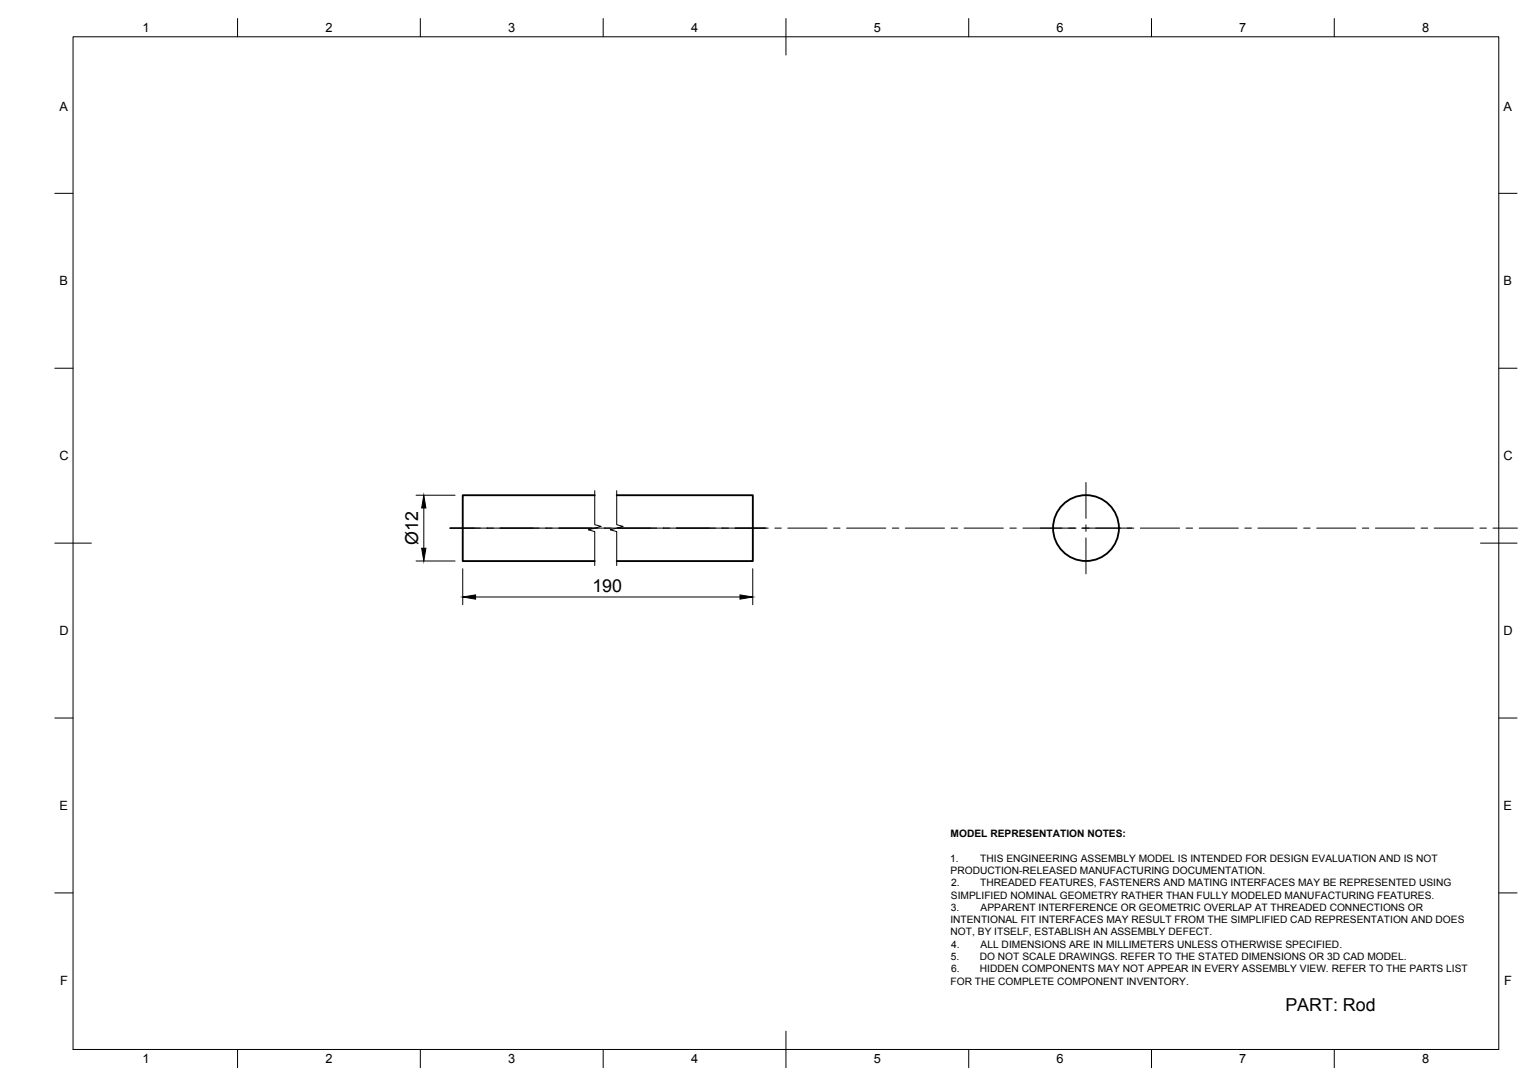
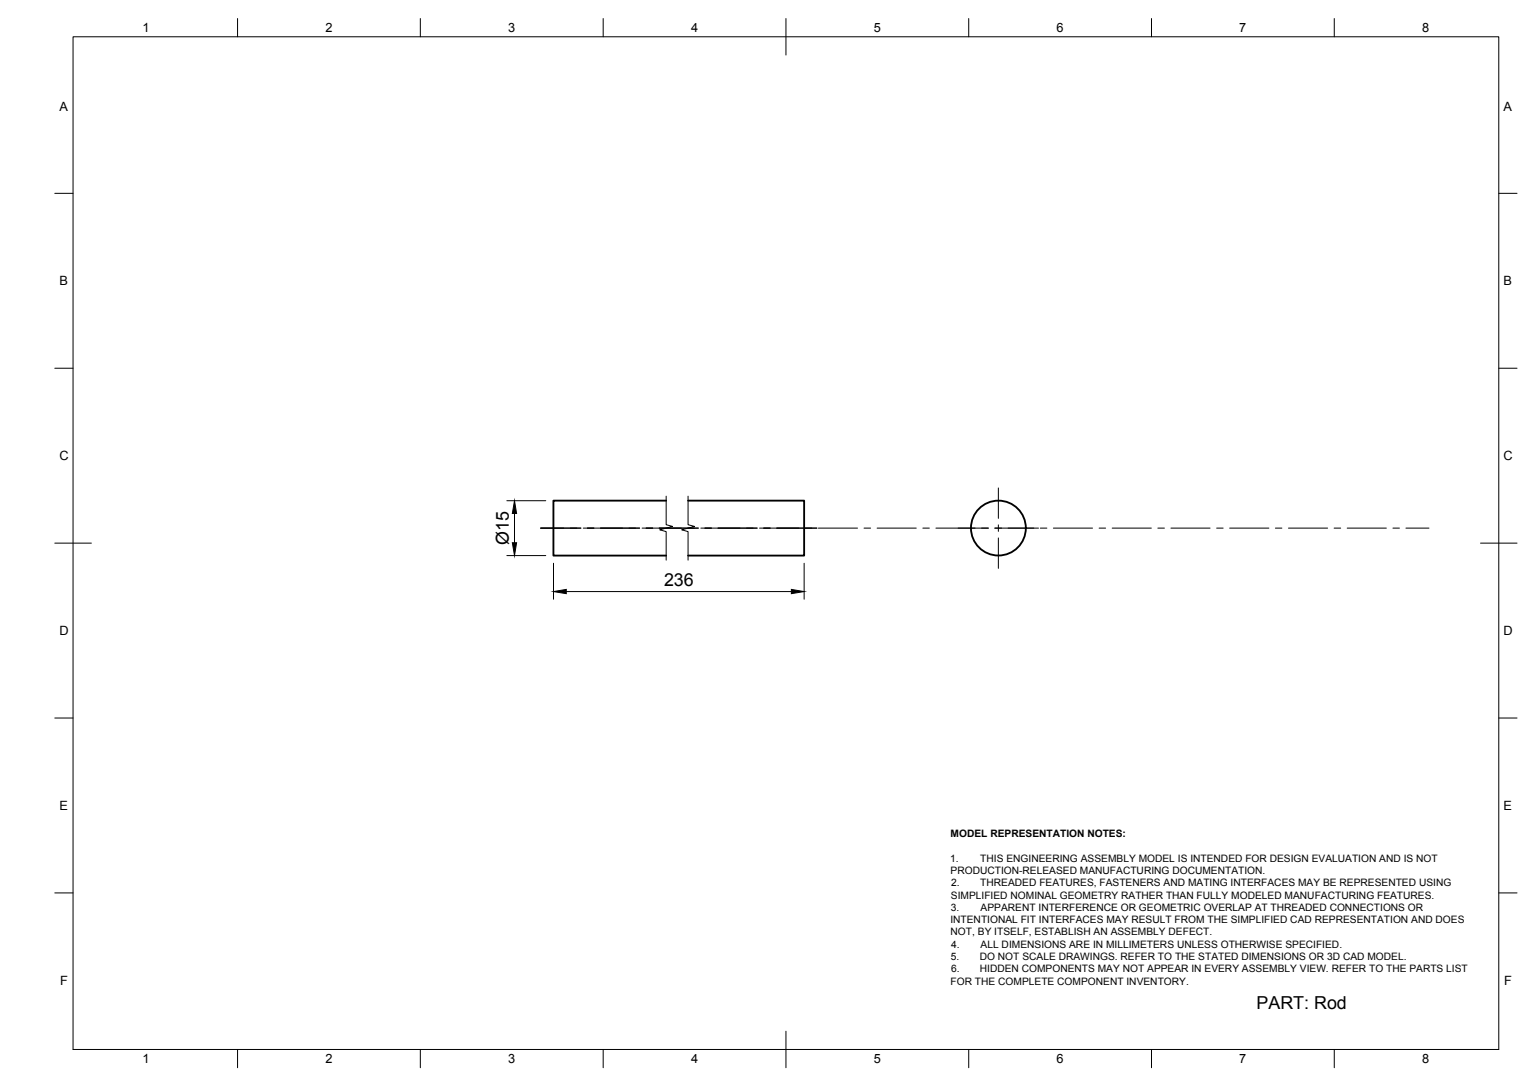
ISO-10303-21;
HEADER;
/* Generated by software containing ST-Developer
 * from STEP Tools, Inc. (www.steptools.com) 
 */

FILE_DESCRIPTION(
/* description */ (''),
/* implementation_level */ '2;1');

FILE_NAME(
/* name */ 'Rod.step',
/* time_stamp */ '2026-10-05T15:35:09-07:00',
/* author */ (''),
/* organization */ (''),
/* preprocessor_version */ 'ST-DEVELOPER v20.2',
/* originating_system */ 'Autodesk Translation Framework v15.15.0.0',
/* authorisation */ '');

FILE_SCHEMA (('AUTOMOTIVE_DESIGN { 1 0 10303 214 3 1 1 }'));
ENDSEC;

DATA;
#10=MECHANICAL_DESIGN_GEOMETRIC_PRESENTATION_REPRESENTATION('',(#550),#74523);
#532=SHAPE_REPRESENTATION_RELATIONSHIP('SRR','None',#74565,#541);
#541=ADVANCED_BREP_SHAPE_REPRESENTATION('',(#559),#74521);
#550=STYLED_ITEM('',(#74612),#559);
#559=MANIFOLD_SOLID_BREP('Body1',#4729);
#670=PLANE('',#5064);
#671=PLANE('',#5068);
#808=FACE_OUTER_BOUND('',#998,.T.);
#809=FACE_OUTER_BOUND('',#999,.T.);
#810=FACE_OUTER_BOUND('',#1000,.T.);
#998=EDGE_LOOP('',(#3612));
#999=EDGE_LOOP('',(#3613,#3614,#3615,#3616));
#1000=EDGE_LOOP('',(#3617));
#1195=LINE('',#7979,#1392);
#1392=VECTOR('',#5749,7.5);
#1514=CIRCLE('',#5065,7.5);
#1515=CIRCLE('',#5067,7.5);
#1741=VERTEX_POINT('',#7974);
#1742=VERTEX_POINT('',#7977);
#2507=EDGE_CURVE('',#1741,#1741,#1514,.T.);
#2508=EDGE_CURVE('',#1742,#1742,#1515,.T.);
#2509=EDGE_CURVE('',#1742,#1741,#1195,.T.);
#3612=ORIENTED_EDGE('',*,*,#2507,.T.);
#3613=ORIENTED_EDGE('',*,*,#2508,.F.);
#3614=ORIENTED_EDGE('',*,*,#2509,.T.);
#3615=ORIENTED_EDGE('',*,*,#2507,.F.);
#3616=ORIENTED_EDGE('',*,*,#2509,.F.);
#3617=ORIENTED_EDGE('',*,*,#2508,.T.);
#4574=CYLINDRICAL_SURFACE('',#5066,7.5);
#4704=ADVANCED_FACE('',(#808),#670,.F.);
#4705=ADVANCED_FACE('',(#809),#4574,.T.);
#4706=ADVANCED_FACE('',(#810),#671,.T.);
#4729=CLOSED_SHELL('',(#4704,#4705,#4706));
#5063=AXIS2_PLACEMENT_3D('',#7972,#5739,#5740);
#5064=AXIS2_PLACEMENT_3D('',#7973,#5741,#5742);
#5065=AXIS2_PLACEMENT_3D('',#7975,#5743,#5744);
#5066=AXIS2_PLACEMENT_3D('',#7976,#5745,#5746);
#5067=AXIS2_PLACEMENT_3D('',#7978,#5747,#5748);
#5068=AXIS2_PLACEMENT_3D('',#7980,#5750,#5751);
#5739=DIRECTION('axis',(0.,0.,1.));
#5740=DIRECTION('refdir',(1.,0.,0.));
#5741=DIRECTION('center_axis',(0.,1.,0.));
#5742=DIRECTION('ref_axis',(1.,0.,0.));
#5743=DIRECTION('center_axis',(0.,-1.,0.));
#5744=DIRECTION('ref_axis',(1.,0.,0.));
#5745=DIRECTION('center_axis',(0.,1.,0.));
#5746=DIRECTION('ref_axis',(1.,0.,0.));
#5747=DIRECTION('center_axis',(0.,1.,0.));
#5748=DIRECTION('ref_axis',(1.,0.,0.));
#5749=DIRECTION('',(0.,-1.,0.));
#5750=DIRECTION('center_axis',(0.,1.,0.));
#5751=DIRECTION('ref_axis',(1.,0.,0.));
#7972=CARTESIAN_POINT('',(0.,0.,0.));
#7973=CARTESIAN_POINT('Origin',(175.231676812499,-118.,15.));
#7974=CARTESIAN_POINT('',(167.731676812499,-118.,15.));
#7975=CARTESIAN_POINT('Origin',(175.231676812499,-118.,15.));
#7976=CARTESIAN_POINT('Origin',(175.231676812499,0.,15.));
#7977=CARTESIAN_POINT('',(167.731676812499,118.,15.));
#7978=CARTESIAN_POINT('Origin',(175.231676812499,118.,15.));
#7979=CARTESIAN_POINT('',(167.731676812499,0.,15.));
#7980=CARTESIAN_POINT('Origin',(175.231676812499,118.,15.));
#74510=UNCERTAINTY_MEASURE_WITH_UNIT(LENGTH_MEASURE(0.01),#74524,
'DISTANCE_ACCURACY_VALUE',
'Maximum model space distance between geometric entities at asserted c
onnectivities');
#74512=UNCERTAINTY_MEASURE_WITH_UNIT(LENGTH_MEASURE(0.01),#74524,
'DISTANCE_ACCURACY_VALUE',
'Maximum model space distance between geometric entities at asserted c
onnectivities');
#74521=(
GEOMETRIC_REPRESENTATION_CONTEXT(3)
GLOBAL_UNCERTAINTY_ASSIGNED_CONTEXT((#74510))
GLOBAL_UNIT_ASSIGNED_CONTEXT((#74524,#74526,#74527))
REPRESENTATION_CONTEXT('','3D')
);
#74523=(
GEOMETRIC_REPRESENTATION_CONTEXT(3)
GLOBAL_UNCERTAINTY_ASSIGNED_CONTEXT((#74512))
GLOBAL_UNIT_ASSIGNED_CONTEXT((#74524,#74526,#74527))
REPRESENTATION_CONTEXT('','3D')
);
#74524=(
LENGTH_UNIT()
NAMED_UNIT(*)
SI_UNIT(.MILLI.,.METRE.)
);
#74526=(
NAMED_UNIT(*)
PLANE_ANGLE_UNIT()
SI_UNIT($,.RADIAN.)
);
#74527=(
NAMED_UNIT(*)
SI_UNIT($,.STERADIAN.)
SOLID_ANGLE_UNIT()
);
#74536=SHAPE_DEFINITION_REPRESENTATION(#74546,#74565);
#74546=PRODUCT_DEFINITION_SHAPE('',$,#74576);
#74565=SHAPE_REPRESENTATION('',(#5063),#74521);
#74567=PRODUCT_DEFINITION_CONTEXT('part definition',#74599,'design');
#74576=PRODUCT_DEFINITION('Rod','Rod',#74586,#74567);
#74586=PRODUCT_DEFINITION_FORMATION('',$,#74609);
#74599=APPLICATION_CONTEXT(
'Core Data for Automotive Mechanical Design Process');
#74600=PRODUCT_CONTEXT('part definition',#74599,'mechanical');
#74609=PRODUCT('Rod','Rod',$,(#74600));
#74612=PRESENTATION_STYLE_ASSIGNMENT((#74615));
#74615=SURFACE_STYLE_USAGE(.BOTH.,#74618);
#74618=SURFACE_SIDE_STYLE('',(#74621));
#74621=SURFACE_STYLE_FILL_AREA(#74624);
#74624=FILL_AREA_STYLE('Opaque(215,0,0)',(#74627));
#74627=FILL_AREA_STYLE_COLOUR('Opaque(215,0,0)',#74630);
#74630=COLOUR_RGB('Opaque(215,0,0)', 0.09019608, 0.27058824, 0.51372549);
ENDSEC;
END-ISO-10303-21;
